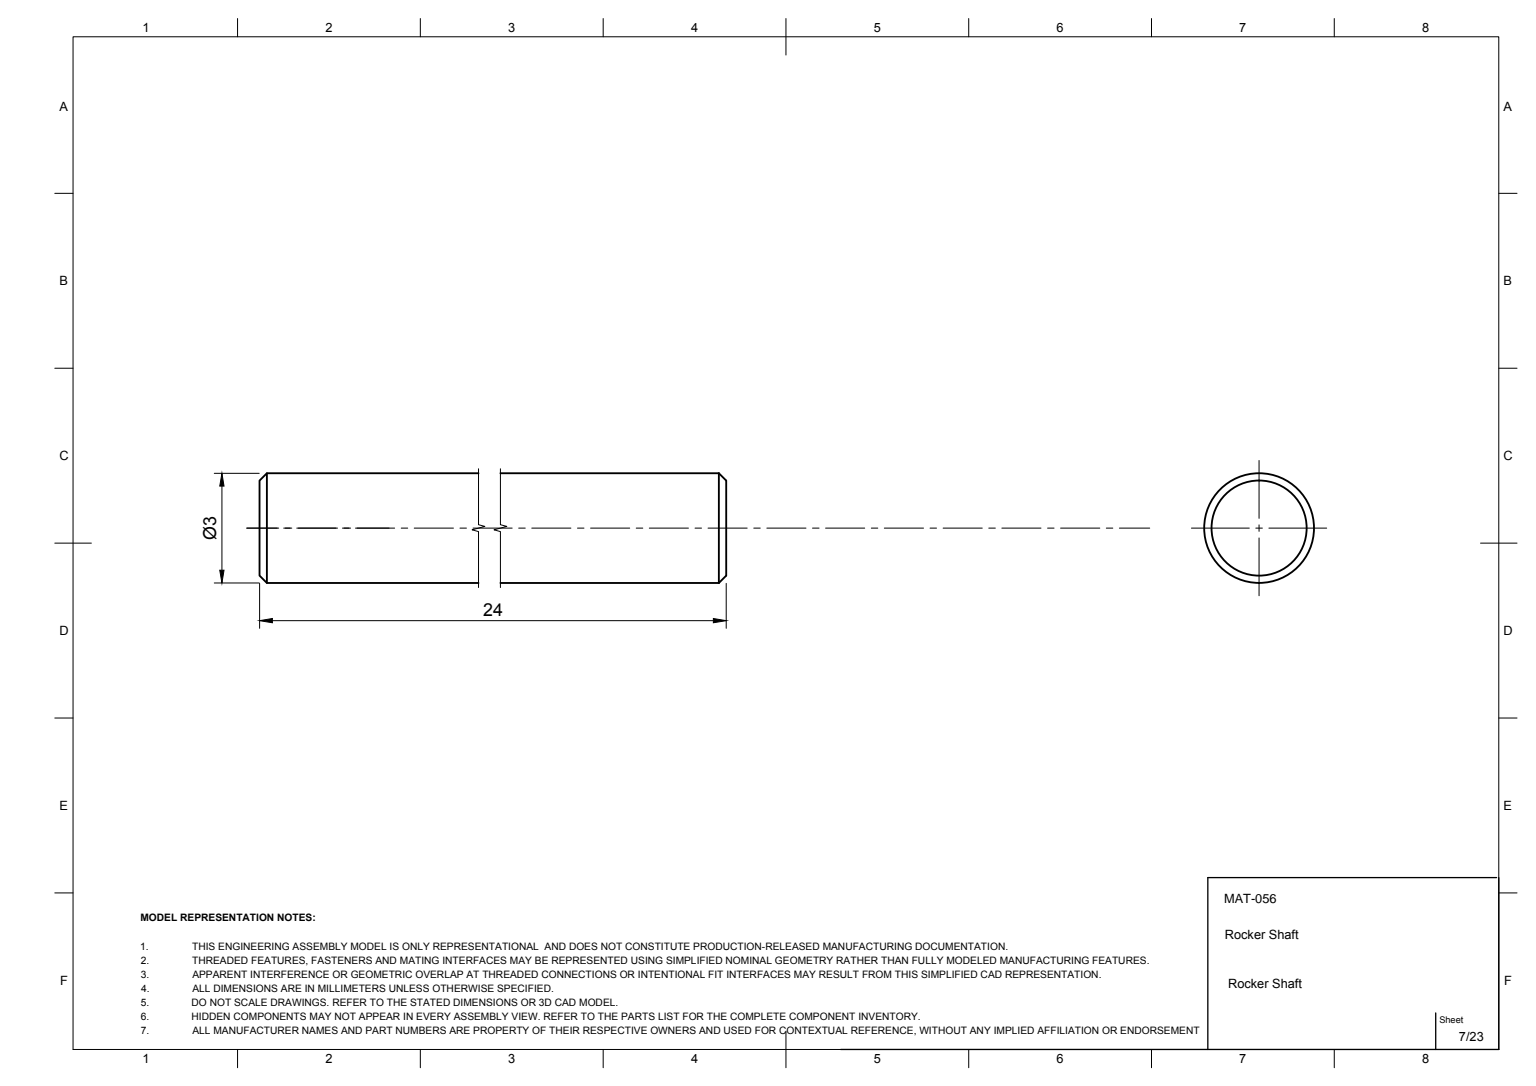
ISO-10303-21;
HEADER;
/* Generated by software containing ST-Developer
 * from STEP Tools, Inc. (www.steptools.com) 
 */

FILE_DESCRIPTION(
/* description */ (''),
/* implementation_level */ '2;1');

FILE_NAME(
/* name */ 'Rocker Shaft.step',
/* time_stamp */ '2026-10-28T16:47:13+01:00',
/* author */ (''),
/* organization */ (''),
/* preprocessor_version */ 'ST-DEVELOPER v20.2',
/* originating_system */ 'Autodesk Translation Framework v15.17.0.0',
/* authorisation */ '');

FILE_SCHEMA (('AUTOMOTIVE_DESIGN { 1 0 10303 214 3 1 1 }'));
ENDSEC;

DATA;
#10=MECHANICAL_DESIGN_GEOMETRIC_PRESENTATION_REPRESENTATION('',(#4572),#459242);
#4409=SHAPE_REPRESENTATION_RELATIONSHIP('SRR','None',#459334,#4430);
#4430=ADVANCED_BREP_SHAPE_REPRESENTATION('',(#4452),#459223);
#4452=MANIFOLD_SOLID_BREP('Shaft body',#94630);
#4572=STYLED_ITEM('',(#459526),#4452);
#4708=CONICAL_SURFACE('',#97224,1.4,0.785398163397448);
#4709=CONICAL_SURFACE('',#97230,1.4,0.785398163397448);
#5587=PLANE('',#97229);
#5588=PLANE('',#97232);
#7430=FACE_OUTER_BOUND('',#13295,.T.);
#7431=FACE_OUTER_BOUND('',#13296,.T.);
#7432=FACE_OUTER_BOUND('',#13297,.T.);
#7433=FACE_OUTER_BOUND('',#13298,.T.);
#7434=FACE_OUTER_BOUND('',#13299,.T.);
#13295=EDGE_LOOP('',(#63806,#63807,#63808,#63809));
#13296=EDGE_LOOP('',(#63810,#63811,#63812,#63813));
#13297=EDGE_LOOP('',(#63814));
#13298=EDGE_LOOP('',(#63815,#63816,#63817,#63818));
#13299=EDGE_LOOP('',(#63819));
#19456=CIRCLE('',#97225,1.3);
#19457=CIRCLE('',#97226,1.5);
#19458=CIRCLE('',#97228,1.5);
#19459=CIRCLE('',#97231,1.3);
#28284=LINE('',#145844,#32086);
#28285=LINE('',#145848,#32087);
#28286=LINE('',#145854,#32088);
#32086=VECTOR('',#111456,1.4);
#32087=VECTOR('',#111461,1.5);
#32088=VECTOR('',#111470,1.4);
#36488=VERTEX_POINT('',#145841);
#36489=VERTEX_POINT('',#145843);
#36490=VERTEX_POINT('',#145847);
#36491=VERTEX_POINT('',#145852);
#46405=EDGE_CURVE('',#36488,#36488,#19456,.T.);
#46406=EDGE_CURVE('',#36488,#36489,#28284,.T.);
#46407=EDGE_CURVE('',#36489,#36489,#19457,.T.);
#46408=EDGE_CURVE('',#36489,#36490,#28285,.T.);
#46409=EDGE_CURVE('',#36490,#36490,#19458,.T.);
#46410=EDGE_CURVE('',#36491,#36491,#19459,.T.);
#46411=EDGE_CURVE('',#36491,#36490,#28286,.T.);
#63806=ORIENTED_EDGE('',*,*,#46405,.T.);
#63807=ORIENTED_EDGE('',*,*,#46406,.T.);
#63808=ORIENTED_EDGE('',*,*,#46407,.T.);
#63809=ORIENTED_EDGE('',*,*,#46406,.F.);
#63810=ORIENTED_EDGE('',*,*,#46407,.F.);
#63811=ORIENTED_EDGE('',*,*,#46408,.T.);
#63812=ORIENTED_EDGE('',*,*,#46409,.F.);
#63813=ORIENTED_EDGE('',*,*,#46408,.F.);
#63814=ORIENTED_EDGE('',*,*,#46405,.F.);
#63815=ORIENTED_EDGE('',*,*,#46410,.T.);
#63816=ORIENTED_EDGE('',*,*,#46411,.T.);
#63817=ORIENTED_EDGE('',*,*,#46409,.T.);
#63818=ORIENTED_EDGE('',*,*,#46411,.F.);
#63819=ORIENTED_EDGE('',*,*,#46410,.F.);
#87524=CYLINDRICAL_SURFACE('',#97227,1.5);
#89894=ADVANCED_FACE('',(#7430),#4708,.T.);
#89895=ADVANCED_FACE('',(#7431),#87524,.T.);
#89896=ADVANCED_FACE('',(#7432),#5587,.F.);
#89897=ADVANCED_FACE('',(#7433),#4709,.T.);
#89898=ADVANCED_FACE('',(#7434),#5588,.T.);
#94630=CLOSED_SHELL('',(#89894,#89895,#89896,#89897,#89898));
#97223=AXIS2_PLACEMENT_3D('',#145839,#111450,#111451);
#97224=AXIS2_PLACEMENT_3D('',#145840,#111452,#111453);
#97225=AXIS2_PLACEMENT_3D('',#145842,#111454,#111455);
#97226=AXIS2_PLACEMENT_3D('',#145845,#111457,#111458);
#97227=AXIS2_PLACEMENT_3D('',#145846,#111459,#111460);
#97228=AXIS2_PLACEMENT_3D('',#145849,#111462,#111463);
#97229=AXIS2_PLACEMENT_3D('',#145850,#111464,#111465);
#97230=AXIS2_PLACEMENT_3D('',#145851,#111466,#111467);
#97231=AXIS2_PLACEMENT_3D('',#145853,#111468,#111469);
#97232=AXIS2_PLACEMENT_3D('',#145855,#111471,#111472);
#111450=DIRECTION('axis',(0.,0.,1.));
#111451=DIRECTION('refdir',(1.,0.,0.));
#111452=DIRECTION('center_axis',(-1.17238944502697E-33,1.22459810574157E-16,
1.));
#111453=DIRECTION('ref_axis',(-1.,-1.07747590158145E-32,8.53125817097821E-20));
#111454=DIRECTION('center_axis',(1.83750175990301E-19,1.22464679914735E-16,
1.));
#111455=DIRECTION('ref_axis',(-1.,-1.07627038873394E-32,1.83750175990301E-19));
#111456=DIRECTION('',(0.707106781186548,-3.4431437427623E-21,0.707106781186548));
#111457=DIRECTION('center_axis',(-1.83750175990301E-19,-1.22464679914735E-16,
-1.));
#111458=DIRECTION('ref_axis',(-1.,-1.07852067938263E-32,-1.17238944502697E-33));
#111459=DIRECTION('center_axis',(1.17238944502697E-33,-1.22459810574157E-16,
-1.));
#111460=DIRECTION('ref_axis',(-1.,-1.07852067938263E-32,-1.17238944502697E-33));
#111461=DIRECTION('',(-1.17238944502697E-33,1.22459810574157E-16,1.));
#111462=DIRECTION('center_axis',(1.83750175990301E-19,1.22464679914735E-16,
1.));
#111463=DIRECTION('ref_axis',(-1.,-1.07852067938263E-32,-1.17238944502697E-33));
#111464=DIRECTION('center_axis',(1.83750175990301E-19,1.22464679914735E-16,
1.));
#111465=DIRECTION('ref_axis',(-1.,-1.07627047820816E-32,1.83750175990301E-19));
#111466=DIRECTION('center_axis',(1.17238944502697E-33,-1.22459810574157E-16,
-1.));
#111467=DIRECTION('ref_axis',(-1.,-1.07747590158145E-32,8.53125817097821E-20));
#111468=DIRECTION('center_axis',(-1.83750175990301E-19,-1.22464679914735E-16,
-1.));
#111469=DIRECTION('ref_axis',(-1.,-1.07627038873394E-32,1.83750175990301E-19));
#111470=DIRECTION('',(0.707106781186548,3.4431437427623E-21,-0.707106781186548));
#111471=DIRECTION('center_axis',(1.83750175990301E-19,1.22464679914735E-16,
1.));
#111472=DIRECTION('ref_axis',(-1.,-1.07627047820816E-32,1.83750175990301E-19));
#145839=CARTESIAN_POINT('',(0.,0.,0.));
#145840=CARTESIAN_POINT('Origin',(4.44089209850063E-15,0.,0.1));
#145841=CARTESIAN_POINT('',(1.30000000000001,0.,0.));
#145842=CARTESIAN_POINT('Origin',(4.44089209850063E-15,0.,0.));
#145843=CARTESIAN_POINT('',(1.50000000000001,0.,0.2));
#145844=CARTESIAN_POINT('',(1.40000000000001,-1.7145055188063E-16,0.1));
#145845=CARTESIAN_POINT('Origin',(4.44089209850063E-15,0.,0.2));
#145846=CARTESIAN_POINT('Origin',(4.44089209850063E-15,2.22044604925031E-15,
24.));
#145847=CARTESIAN_POINT('',(1.50000000000001,2.22044604925031E-15,23.8));
#145848=CARTESIAN_POINT('',(1.50000000000001,2.03674902937821E-15,24.));
#145849=CARTESIAN_POINT('Origin',(4.44089209850063E-15,2.22044604925031E-15,
23.8));
#145850=CARTESIAN_POINT('Origin',(4.44089209850063E-15,0.,0.));
#145851=CARTESIAN_POINT('Origin',(4.44089209850063E-15,2.22044604925031E-15,
23.9));
#145852=CARTESIAN_POINT('',(1.30000000000001,2.22044604925031E-15,24.));
#145853=CARTESIAN_POINT('Origin',(4.44089209850063E-15,2.22044604925031E-15,
24.));
#145854=CARTESIAN_POINT('',(1.40000000000001,2.39189660113094E-15,23.9));
#145855=CARTESIAN_POINT('Origin',(4.44089209850063E-15,2.22044604925031E-15,
24.));
#459197=UNCERTAINTY_MEASURE_WITH_UNIT(LENGTH_MEASURE(0.01),#459243,
'DISTANCE_ACCURACY_VALUE',
'Maximum model space distance between geometric entities at asserted c
onnectivities');
#459216=UNCERTAINTY_MEASURE_WITH_UNIT(LENGTH_MEASURE(0.01),#459243,
'DISTANCE_ACCURACY_VALUE',
'Maximum model space distance between geometric entities at asserted c
onnectivities');
#459223=(
GEOMETRIC_REPRESENTATION_CONTEXT(3)
GLOBAL_UNCERTAINTY_ASSIGNED_CONTEXT((#459197))
GLOBAL_UNIT_ASSIGNED_CONTEXT((#459243,#459245,#459246))
REPRESENTATION_CONTEXT('','3D')
);
#459242=(
GEOMETRIC_REPRESENTATION_CONTEXT(3)
GLOBAL_UNCERTAINTY_ASSIGNED_CONTEXT((#459216))
GLOBAL_UNIT_ASSIGNED_CONTEXT((#459243,#459245,#459246))
REPRESENTATION_CONTEXT('','3D')
);
#459243=(
LENGTH_UNIT()
NAMED_UNIT(*)
SI_UNIT(.MILLI.,.METRE.)
);
#459245=(
NAMED_UNIT(*)
PLANE_ANGLE_UNIT()
SI_UNIT($,.RADIAN.)
);
#459246=(
NAMED_UNIT(*)
SI_UNIT($,.STERADIAN.)
SOLID_ANGLE_UNIT()
);
#459253=SHAPE_DEFINITION_REPRESENTATION(#459278,#459334);
#459278=PRODUCT_DEFINITION_SHAPE('',$,#459360);
#459334=SHAPE_REPRESENTATION('',(#97223),#459223);
#459353=PRODUCT_DEFINITION_CONTEXT('part definition',#459430,'design');
#459360=PRODUCT_DEFINITION('Rocker Shaft','Rocker Shaft',#459385,#459353);
#459385=PRODUCT_DEFINITION_FORMATION('',$,#459438);
#459430=APPLICATION_CONTEXT(
'Core Data for Automotive Mechanical Design Process');
#459431=PRODUCT_CONTEXT('part definition',#459430,'mechanical');
#459438=PRODUCT('Rocker Shaft','Rocker Shaft',$,(#459431));
#459520=COLOUR_RGB('Grey',0.48,0.52,0.57);
#459521=FILL_AREA_STYLE_COLOUR('',#459520);
#459522=FILL_AREA_STYLE('',(#459521));
#459523=SURFACE_STYLE_FILL_AREA(#459522);
#459524=SURFACE_SIDE_STYLE('',(#459523));
#459525=SURFACE_STYLE_USAGE(.BOTH.,#459524);
#459526=PRESENTATION_STYLE_ASSIGNMENT((#459525));
ENDSEC;
END-ISO-10303-21;
